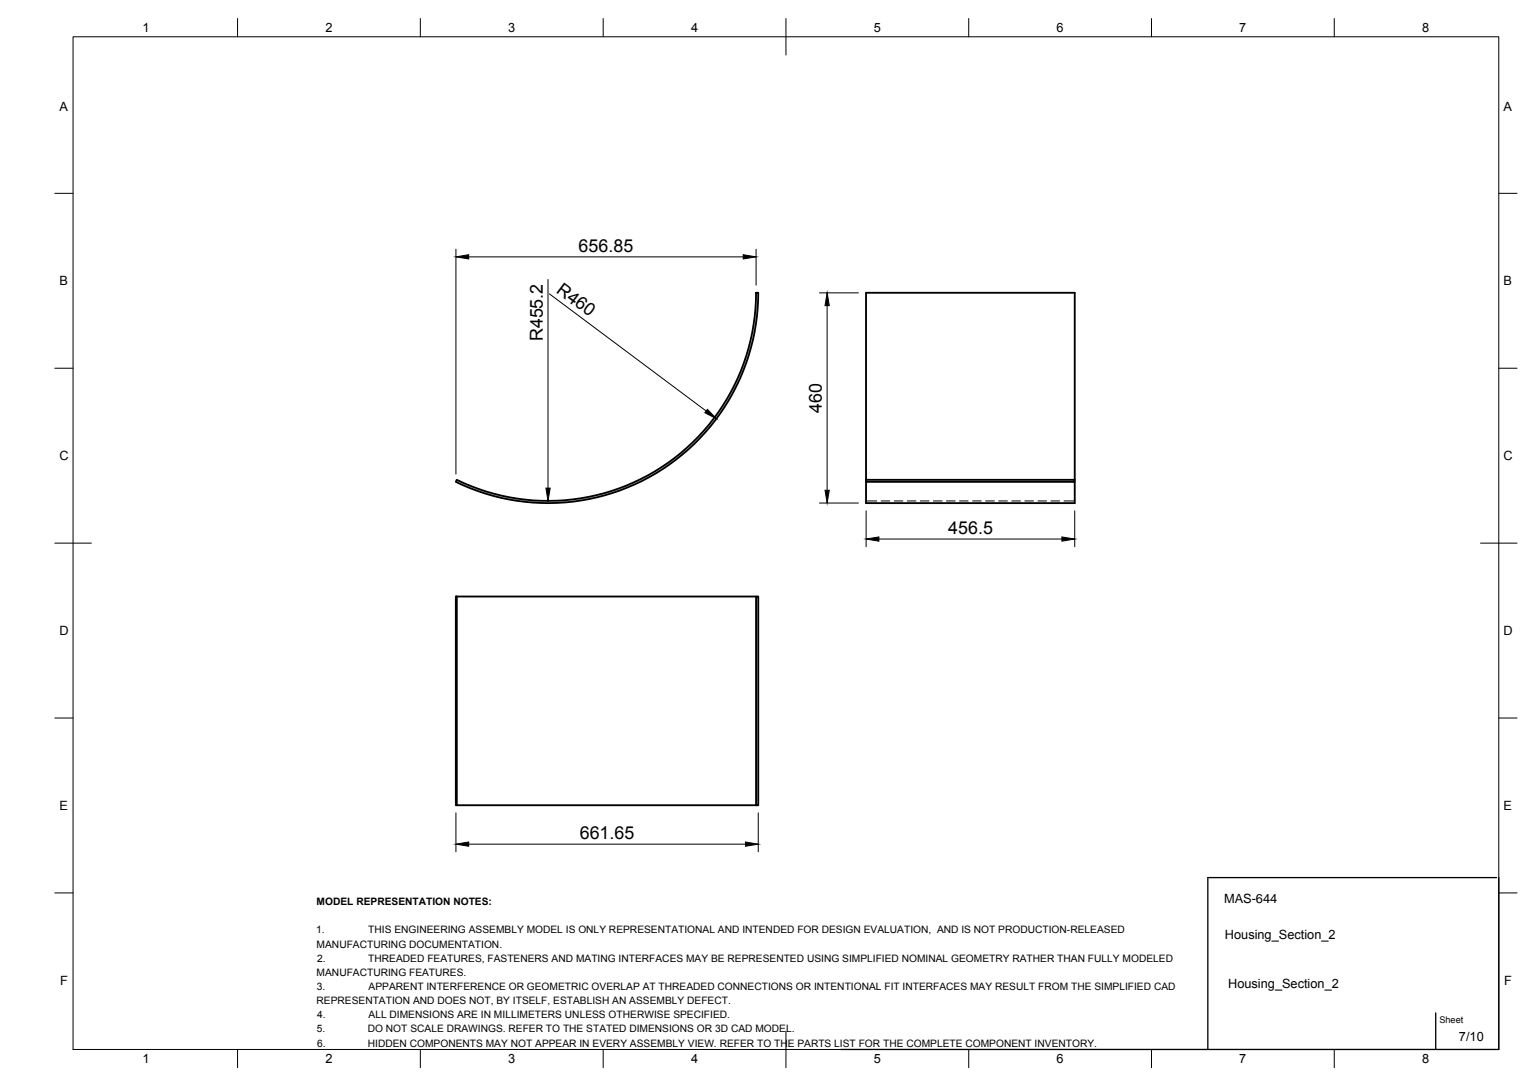
ISO-10303-21;
HEADER;
FILE_DESCRIPTION((''),'2;1');
FILE_NAME('Housing_Section_2.step','2026-10-09T11:38:21-07:00',(''),(''),'','','');
FILE_SCHEMA (('AUTOMOTIVE_DESIGN { 1 0 10303 214 3 1 1 }'));
ENDSEC;
DATA;
#10=MECHANICAL_DESIGN_GEOMETRIC_PRESENTATION_REPRESENTATION('',(#63),#3619);
#47=SHAPE_REPRESENTATION_RELATIONSHIP('SRR','None',#3655,#55) ;
#55=ADVANCED_BREP_SHAPE_REPRESENTATION('',(#71),#3615) ;
#63=STYLED_ITEM('',(#3700),#71) ;
#71=MANIFOLD_SOLID_BREP('Body1',#2087) ;
#187=PLANE('',#2354) ;
#188=PLANE('',#2358) ;
#189=PLANE('',#2362) ;
#190=PLANE('',#2363) ;
#289=FACE_OUTER_BOUND('',#479,.T.) ;
#290=FACE_OUTER_BOUND('',#480,.T.) ;
#291=FACE_OUTER_BOUND('',#481,.T.) ;
#292=FACE_OUTER_BOUND('',#482,.T.) ;
#293=FACE_OUTER_BOUND('',#483,.T.) ;
#294=FACE_OUTER_BOUND('',#484,.T.) ;
#479=EDGE_LOOP('',(#1795,#1796,#1797,#1798)) ;
#480=EDGE_LOOP('',(#1799,#1800,#1801,#1802)) ;
#481=EDGE_LOOP('',(#1803,#1804,#1805,#1806)) ;
#482=EDGE_LOOP('',(#1807,#1808,#1809,#1810)) ;
#483=EDGE_LOOP('',(#1811,#1812,#1813,#1814)) ;
#484=EDGE_LOOP('',(#1815,#1816,#1817,#1818)) ;
#623=LINE('',#3456,#787) ;
#624=LINE('',#3458,#788) ;
#625=LINE('',#3460,#789) ;
#626=LINE('',#3461,#790) ;
#627=LINE('',#3466,#791) ;
#628=LINE('',#3470,#792) ;
#629=LINE('',#3472,#793) ;
#630=LINE('',#3473,#794) ;
#787=VECTOR('',#2871,1000.) ;
#788=VECTOR('',#2872,1000.) ;
#789=VECTOR('',#2873,1000.) ;
#790=VECTOR('',#2874,1000.) ;
#791=VECTOR('',#2879,1000.) ;
#792=VECTOR('',#2884,1000.) ;
#793=VECTOR('',#2885,1000.) ;
#794=VECTOR('',#2886,1000.) ;
#931=CIRCLE('',#2356,460.) ;
#932=CIRCLE('',#2357,460.) ;
#933=CIRCLE('',#2360,455.2) ;
#934=CIRCLE('',#2361,455.2) ;
#1079=VERTEX_POINT('',#3454) ;
#1080=VERTEX_POINT('',#3455) ;
#1081=VERTEX_POINT('',#3457) ;
#1082=VERTEX_POINT('',#3459) ;
#1083=VERTEX_POINT('',#3463) ;
#1084=VERTEX_POINT('',#3465) ;
#1085=VERTEX_POINT('',#3469) ;
#1086=VERTEX_POINT('',#3471) ;
#1323=EDGE_CURVE('',#1079,#1080,#623,.T.) ;
#1324=EDGE_CURVE('',#1081,#1079,#624,.T.) ;
#1325=EDGE_CURVE('',#1081,#1082,#625,.T.) ;
#1326=EDGE_CURVE('',#1082,#1080,#626,.T.) ;
#1327=EDGE_CURVE('',#1083,#1079,#931,.T.) ;
#1328=EDGE_CURVE('',#1084,#1083,#627,.T.) ;
#1329=EDGE_CURVE('',#1084,#1081,#932,.T.) ;
#1330=EDGE_CURVE('',#1085,#1083,#628,.T.) ;
#1331=EDGE_CURVE('',#1086,#1085,#629,.T.) ;
#1332=EDGE_CURVE('',#1086,#1084,#630,.T.) ;
#1333=EDGE_CURVE('',#1085,#1080,#933,.T.) ;
#1334=EDGE_CURVE('',#1086,#1082,#934,.T.) ;
#1795=ORIENTED_EDGE('',*,*,#1323,.F.) ;
#1796=ORIENTED_EDGE('',*,*,#1324,.F.) ;
#1797=ORIENTED_EDGE('',*,*,#1325,.T.) ;
#1798=ORIENTED_EDGE('',*,*,#1326,.T.) ;
#1799=ORIENTED_EDGE('',*,*,#1327,.F.) ;
#1800=ORIENTED_EDGE('',*,*,#1328,.F.) ;
#1801=ORIENTED_EDGE('',*,*,#1329,.T.) ;
#1802=ORIENTED_EDGE('',*,*,#1324,.T.) ;
#1803=ORIENTED_EDGE('',*,*,#1330,.F.) ;
#1804=ORIENTED_EDGE('',*,*,#1331,.F.) ;
#1805=ORIENTED_EDGE('',*,*,#1332,.T.) ;
#1806=ORIENTED_EDGE('',*,*,#1328,.T.) ;
#1807=ORIENTED_EDGE('',*,*,#1333,.T.) ;
#1808=ORIENTED_EDGE('',*,*,#1326,.F.) ;
#1809=ORIENTED_EDGE('',*,*,#1334,.F.) ;
#1810=ORIENTED_EDGE('',*,*,#1331,.T.) ;
#1811=ORIENTED_EDGE('',*,*,#1334,.T.) ;
#1812=ORIENTED_EDGE('',*,*,#1325,.F.) ;
#1813=ORIENTED_EDGE('',*,*,#1329,.F.) ;
#1814=ORIENTED_EDGE('',*,*,#1332,.F.) ;
#1815=ORIENTED_EDGE('',*,*,#1323,.T.) ;
#1816=ORIENTED_EDGE('',*,*,#1333,.F.) ;
#1817=ORIENTED_EDGE('',*,*,#1330,.T.) ;
#1818=ORIENTED_EDGE('',*,*,#1327,.T.) ;
#1969=CYLINDRICAL_SURFACE('',#2355,460.) ;
#1970=CYLINDRICAL_SURFACE('',#2359,455.2) ;
#2051=ADVANCED_FACE('',(#289),#187,.T.) ;
#2052=ADVANCED_FACE('',(#290),#1969,.T.) ;
#2053=ADVANCED_FACE('',(#291),#188,.T.) ;
#2054=ADVANCED_FACE('',(#292),#1970,.F.) ;
#2055=ADVANCED_FACE('',(#293),#189,.T.) ;
#2056=ADVANCED_FACE('',(#294),#190,.F.) ;
#2087=CLOSED_SHELL('',(#2051,#2052,#2053,#2054,#2055,#2056)) ;
#2353=AXIS2_PLACEMENT_3D('',#3452,#2867,#2868) ;
#2354=AXIS2_PLACEMENT_3D('',#3453,#2869,#2870) ;
#2355=AXIS2_PLACEMENT_3D('',#3462,#2875,#2876) ;
#2356=AXIS2_PLACEMENT_3D('',#3464,#2877,#2878) ;
#2357=AXIS2_PLACEMENT_3D('',#3467,#2880,#2881) ;
#2358=AXIS2_PLACEMENT_3D('',#3468,#2882,#2883) ;
#2359=AXIS2_PLACEMENT_3D('',#3474,#2887,#2888) ;
#2360=AXIS2_PLACEMENT_3D('',#3475,#2889,#2890) ;
#2361=AXIS2_PLACEMENT_3D('',#3476,#2891,#2892) ;
#2362=AXIS2_PLACEMENT_3D('',#3477,#2893,#2894) ;
#2363=AXIS2_PLACEMENT_3D('',#3478,#2895,#2896) ;
#2867=DIRECTION('axis',(0.,0.,1.)) ;
#2868=DIRECTION('refdir',(1.,0.,0.)) ;
#2869=DIRECTION('center_axis',(0.898794046299161,-0.438371146789089,0.)) ;
#2870=DIRECTION('ref_axis',(0.438371146789089,0.898794046299161,0.)) ;
#2871=DIRECTION('',(-0.438371146789089,-0.898794046299161,0.)) ;
#2872=DIRECTION('',(0.,0.,-1.)) ;
#2873=DIRECTION('',(-0.438371146789089,-0.898794046299161,0.)) ;
#2874=DIRECTION('',(0.,0.,-1.)) ;
#2875=DIRECTION('center_axis',(0.,0.,-1.)) ;
#2876=DIRECTION('ref_axis',(-1.,0.,0.)) ;
#2877=DIRECTION('center_axis',(0.,0.,-1.)) ;
#2878=DIRECTION('ref_axis',(-1.,0.,0.)) ;
#2879=DIRECTION('',(0.,0.,-1.)) ;
#2880=DIRECTION('center_axis',(0.,0.,-1.)) ;
#2881=DIRECTION('ref_axis',(-1.,0.,0.)) ;
#2882=DIRECTION('center_axis',(1.1613733811914E-14,-1.,0.)) ;
#2883=DIRECTION('ref_axis',(1.,1.1613733811914E-14,0.)) ;
#2884=DIRECTION('',(-1.,-1.1613733811914E-14,0.)) ;
#2885=DIRECTION('',(0.,0.,-1.)) ;
#2886=DIRECTION('',(-1.,-1.1613733811914E-14,0.)) ;
#2887=DIRECTION('center_axis',(0.,0.,-1.)) ;
#2888=DIRECTION('ref_axis',(-1.,0.,0.)) ;
#2889=DIRECTION('center_axis',(0.,0.,-1.)) ;
#2890=DIRECTION('ref_axis',(1.,0.,0.)) ;
#2891=DIRECTION('center_axis',(0.,0.,-1.)) ;
#2892=DIRECTION('ref_axis',(1.,0.,0.)) ;
#2893=DIRECTION('center_axis',(0.,0.,1.)) ;
#2894=DIRECTION('ref_axis',(1.,0.,0.)) ;
#2895=DIRECTION('center_axis',(0.,0.,1.)) ;
#2896=DIRECTION('ref_axis',(1.,0.,0.)) ;
#3452=CARTESIAN_POINT('',(0.,0.,0.)) ;
#3453=CARTESIAN_POINT('Origin',(-23.3492724770243,413.445261297617,456.5)) ;
#3454=CARTESIAN_POINT('',(-23.3492724770243,413.445261297617,-5.55111512312578E-14)) ;
#3455=CARTESIAN_POINT('',(-25.453453981612,409.131049875381,-5.55111512312578E-14)) ;
#3456=CARTESIAN_POINT('',(-23.3492724770243,413.445261297617,-5.55111512312578E-14)) ;
#3457=CARTESIAN_POINT('',(-23.3492724770243,413.445261297617,456.5)) ;
#3458=CARTESIAN_POINT('',(-23.3492724770243,413.445261297617,456.5)) ;
#3459=CARTESIAN_POINT('',(-25.453453981612,409.131049875381,456.5)) ;
#3460=CARTESIAN_POINT('',(-23.3492724770243,413.445261297617,456.5)) ;
#3461=CARTESIAN_POINT('',(-25.453453981612,409.131049875381,456.5)) ;
#3462=CARTESIAN_POINT('Origin',(-225.,2.51053816426691E-13,456.5)) ;
#3463=CARTESIAN_POINT('',(-685.,2.51053816426691E-13,-5.55111512312578E-14)) ;
#3464=CARTESIAN_POINT('Origin',(-225.,2.51053816426691E-13,-5.55111512312578E-14)) ;
#3465=CARTESIAN_POINT('',(-685.,2.51053816426691E-13,456.5)) ;
#3466=CARTESIAN_POINT('',(-685.,2.51053816426691E-13,456.5)) ;
#3467=CARTESIAN_POINT('Origin',(-225.,2.51053816426691E-13,456.5)) ;
#3468=CARTESIAN_POINT('Origin',(-680.200000000001,3.06799738723879E-13,
456.5)) ;
#3469=CARTESIAN_POINT('',(-680.200000000001,3.06799738723879E-13,-5.55111512312578E-14)) ;
#3470=CARTESIAN_POINT('',(-680.200000000001,3.06799738723879E-13,-5.55111512312578E-14)) ;
#3471=CARTESIAN_POINT('',(-680.200000000001,3.06799738723879E-13,456.5)) ;
#3472=CARTESIAN_POINT('',(-680.200000000001,3.06799738723879E-13,456.5)) ;
#3473=CARTESIAN_POINT('',(-680.200000000001,3.06799738723879E-13,456.5)) ;
#3474=CARTESIAN_POINT('Origin',(-225.,2.51053816426691E-13,456.5)) ;
#3475=CARTESIAN_POINT('Origin',(-225.,2.51053816426691E-13,-5.55111512312578E-14)) ;
#3476=CARTESIAN_POINT('Origin',(-225.,2.51053816426691E-13,456.5)) ;
#3477=CARTESIAN_POINT('Origin',(-225.,2.51053816426691E-13,456.5)) ;
#3478=CARTESIAN_POINT('Origin',(-225.,2.51053816426691E-13,-5.55111512312578E-14)) ;
#3605=UNCERTAINTY_MEASURE_WITH_UNIT(LENGTH_MEASURE(0.01),#3620,
'DISTANCE_ACCURACY_VALUE',
'Maximum model space distance between geometric entities at asserted c
onnectivities') ;
#3609=UNCERTAINTY_MEASURE_WITH_UNIT(LENGTH_MEASURE(0.01),#3620,
'DISTANCE_ACCURACY_VALUE',
'Maximum model space distance between geometric entities at asserted c
onnectivities') ;
#3615=(
GEOMETRIC_REPRESENTATION_CONTEXT(3)
GLOBAL_UNCERTAINTY_ASSIGNED_CONTEXT((#3605))
GLOBAL_UNIT_ASSIGNED_CONTEXT((#3620,#3622,#3623))
REPRESENTATION_CONTEXT('','3D')
) ;
#3619=(
GEOMETRIC_REPRESENTATION_CONTEXT(3)
GLOBAL_UNCERTAINTY_ASSIGNED_CONTEXT((#3609))
GLOBAL_UNIT_ASSIGNED_CONTEXT((#3620,#3622,#3623))
REPRESENTATION_CONTEXT('','3D')
) ;
#3620=(
LENGTH_UNIT()
NAMED_UNIT(*)
SI_UNIT(.MILLI.,.METRE.)
) ;
#3622=(
NAMED_UNIT(*)
PLANE_ANGLE_UNIT()
SI_UNIT($,.RADIAN.)
) ;
#3623=(
NAMED_UNIT(*)
SI_UNIT($,.STERADIAN.)
SOLID_ANGLE_UNIT()
) ;
#3629=SHAPE_DEFINITION_REPRESENTATION(#3638,#3655) ;
#3638=PRODUCT_DEFINITION_SHAPE('',$,#3665) ;
#3655=SHAPE_REPRESENTATION('',(#2353),#3615) ;
#3659=PRODUCT_DEFINITION_CONTEXT('part definition',#3688,'design') ;
#3665=PRODUCT_DEFINITION('Housing_Section_2','Housing_Section_2',#3674,
#3659) ;
#3674=PRODUCT_DEFINITION_FORMATION('',$,#3695) ;
#3688=APPLICATION_CONTEXT(
'Core Data for Automotive Mechanical Design Process') ;
#3689=PRODUCT_CONTEXT('part definition',#3688,'mechanical') ;
#3695=PRODUCT('Housing_Section_2','Housing_Section_2',$,(#3689)) ;
#3700=PRESENTATION_STYLE_ASSIGNMENT((#3702)) ;
#3702=SURFACE_STYLE_USAGE(.BOTH.,#3704) ;
#3704=SURFACE_SIDE_STYLE('',(#3706)) ;
#3706=SURFACE_STYLE_FILL_AREA(#3708) ;
#3708=FILL_AREA_STYLE('Opaque(202,209,238)',(#3710)) ;
#3710=FILL_AREA_STYLE_COLOUR('Opaque(202,209,238)',#3712) ;
#3712=COLOUR_RGB('Opaque(202,209,238)', 0.09019608, 0.27058824, 0.51372549) ;
ENDSEC;
END-ISO-10303-21;
